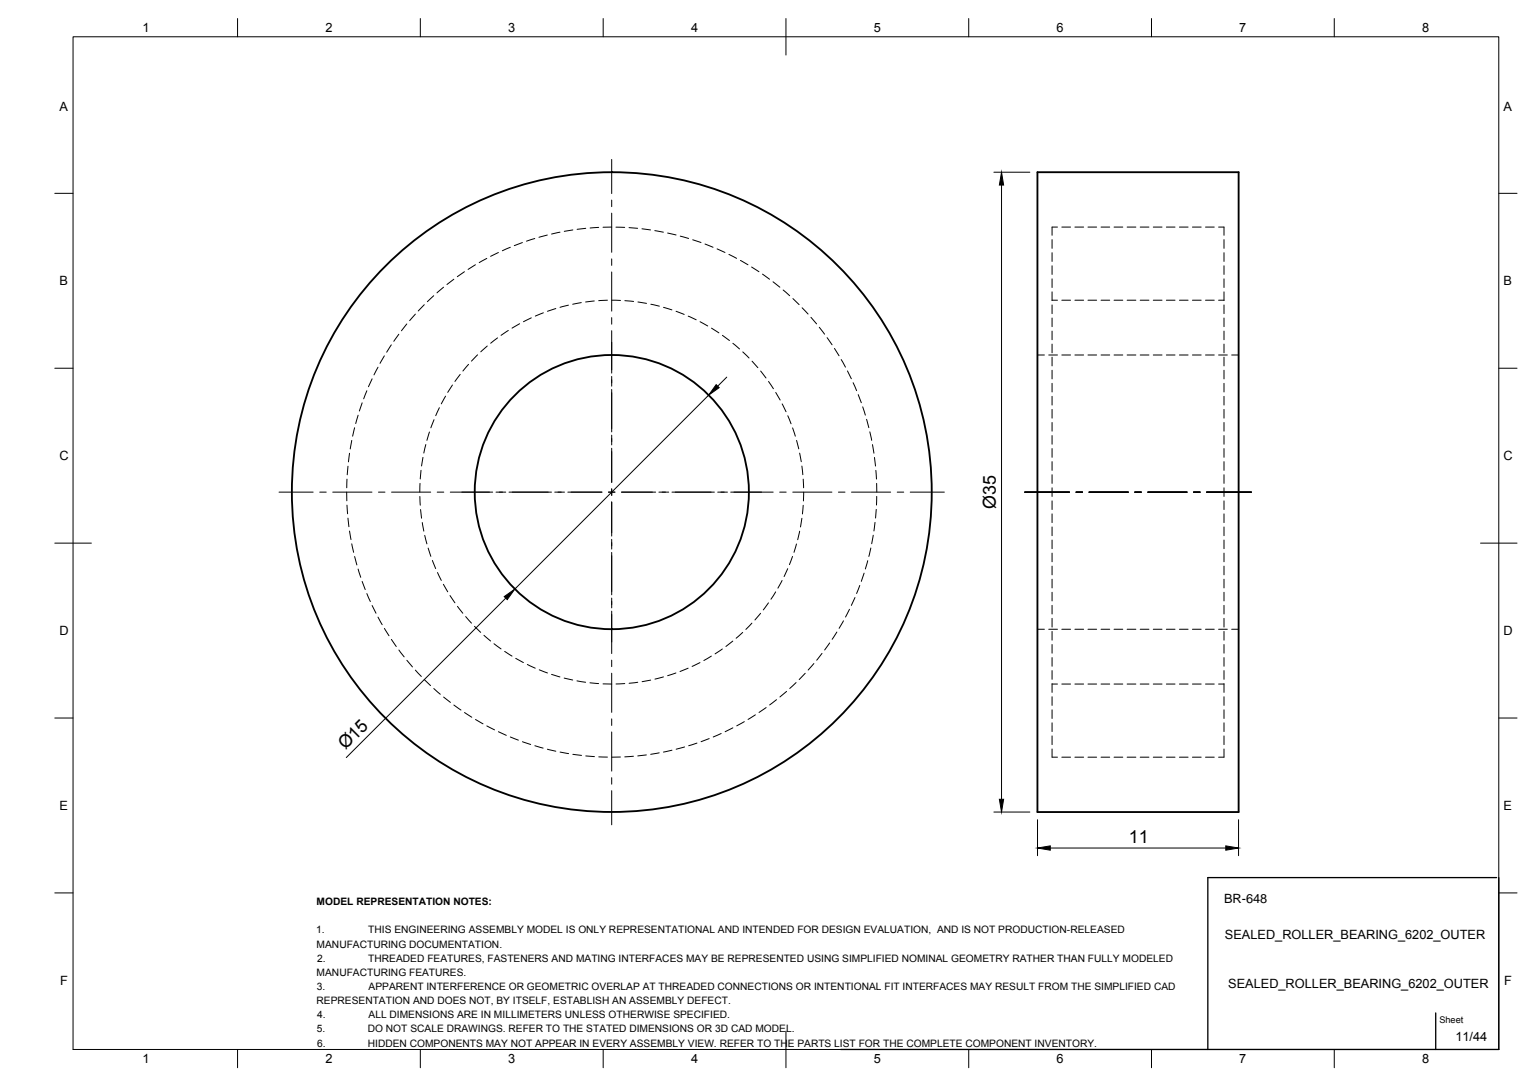
ISO-10303-21;
HEADER;
FILE_DESCRIPTION((''),'2;1');
FILE_NAME('SEALED_ROLLER_BEARING_6202_OUTER.step','2026-10-01T22:05:39-07:00',(''),(''),'','','');
FILE_SCHEMA (('AUTOMOTIVE_DESIGN { 1 0 10303 214 3 1 1 }'));
ENDSEC;
DATA;
#10=MECHANICAL_DESIGN_GEOMETRIC_PRESENTATION_REPRESENTATION('',(#611),#24628);
#485=ORIENTED_CLOSED_SHELL('',*,#13120,.F.) ;
#518=BREP_WITH_VOIDS('SEALED_ROLLER_BEARING_6202_OUTER',#13121,(#485)) ;
#527=SHAPE_REPRESENTATION_RELATIONSHIP('SRR','None',#24799,#569) ;
#569=ADVANCED_BREP_SHAPE_REPRESENTATION('',(#518),#24589) ;
#611=STYLED_ITEM('',(#25034),#518) ;
#839=FACE_BOUND('',#4045,.T.) ;
#840=FACE_BOUND('',#4047,.T.) ;
#841=FACE_BOUND('',#4051,.T.) ;
#842=FACE_BOUND('',#4054,.T.) ;
#1142=LINE('',#20621,#1978) ;
#1143=LINE('',#20623,#1979) ;
#1144=LINE('',#20632,#1980) ;
#1145=LINE('',#20637,#1981) ;
#1978=VECTOR('',#16365,1.05) ;
#1979=VECTOR('',#16368,1.45) ;
#1980=VECTOR('',#16379,1.75) ;
#1981=VECTOR('',#16386,0.75) ;
#2778=CYLINDRICAL_SURFACE('',#14068,1.05) ;
#2779=CYLINDRICAL_SURFACE('',#14069,1.45) ;
#2780=CYLINDRICAL_SURFACE('',#14073,1.75) ;
#2781=CYLINDRICAL_SURFACE('',#14077,0.75) ;
#3124=FACE_OUTER_BOUND('',#4044,.T.) ;
#3125=FACE_OUTER_BOUND('',#4046,.T.) ;
#3126=FACE_OUTER_BOUND('',#4048,.T.) ;
#3127=FACE_OUTER_BOUND('',#4049,.T.) ;
#3128=FACE_OUTER_BOUND('',#4050,.T.) ;
#3129=FACE_OUTER_BOUND('',#4052,.T.) ;
#3130=FACE_OUTER_BOUND('',#4053,.T.) ;
#3131=FACE_OUTER_BOUND('',#4055,.T.) ;
#4044=EDGE_LOOP('',(#9237)) ;
#4045=EDGE_LOOP('',(#9238)) ;
#4046=EDGE_LOOP('',(#9239)) ;
#4047=EDGE_LOOP('',(#9240)) ;
#4048=EDGE_LOOP('',(#9241,#9242,#9243,#9244)) ;
#4049=EDGE_LOOP('',(#9245,#9246,#9247,#9248)) ;
#4050=EDGE_LOOP('',(#9249)) ;
#4051=EDGE_LOOP('',(#9250)) ;
#4052=EDGE_LOOP('',(#9251,#9252,#9253,#9254)) ;
#4053=EDGE_LOOP('',(#9255)) ;
#4054=EDGE_LOOP('',(#9256)) ;
#4055=EDGE_LOOP('',(#9257,#9258,#9259,#9260)) ;
#4980=CIRCLE('',#14063,1.45) ;
#4981=CIRCLE('',#14064,1.05) ;
#4982=CIRCLE('',#14066,1.45) ;
#4983=CIRCLE('',#14067,1.05) ;
#4984=CIRCLE('',#14071,1.75) ;
#4985=CIRCLE('',#14072,0.75) ;
#4986=CIRCLE('',#14074,1.75) ;
#4987=CIRCLE('',#14076,0.75) ;
#5787=VERTEX_POINT('',#20611) ;
#5788=VERTEX_POINT('',#20613) ;
#5789=VERTEX_POINT('',#20616) ;
#5790=VERTEX_POINT('',#20618) ;
#5791=VERTEX_POINT('',#20625) ;
#5792=VERTEX_POINT('',#20627) ;
#5793=VERTEX_POINT('',#20630) ;
#5794=VERTEX_POINT('',#20634) ;
#7108=EDGE_CURVE('',#5787,#5787,#4980,.T.) ;
#7109=EDGE_CURVE('',#5788,#5788,#4981,.T.) ;
#7110=EDGE_CURVE('',#5789,#5789,#4982,.T.) ;
#7111=EDGE_CURVE('',#5790,#5790,#4983,.T.) ;
#7112=EDGE_CURVE('',#5788,#5790,#1142,.T.) ;
#7113=EDGE_CURVE('',#5789,#5787,#1143,.T.) ;
#7114=EDGE_CURVE('',#5791,#5791,#4984,.T.) ;
#7115=EDGE_CURVE('',#5792,#5792,#4985,.T.) ;
#7116=EDGE_CURVE('',#5793,#5793,#4986,.T.) ;
#7117=EDGE_CURVE('',#5793,#5791,#1144,.T.) ;
#7118=EDGE_CURVE('',#5794,#5794,#4987,.T.) ;
#7119=EDGE_CURVE('',#5792,#5794,#1145,.T.) ;
#9237=ORIENTED_EDGE('',*,*,#7108,.F.) ;
#9238=ORIENTED_EDGE('',*,*,#7109,.F.) ;
#9239=ORIENTED_EDGE('',*,*,#7110,.F.) ;
#9240=ORIENTED_EDGE('',*,*,#7111,.F.) ;
#9241=ORIENTED_EDGE('',*,*,#7109,.T.) ;
#9242=ORIENTED_EDGE('',*,*,#7112,.T.) ;
#9243=ORIENTED_EDGE('',*,*,#7111,.T.) ;
#9244=ORIENTED_EDGE('',*,*,#7112,.F.) ;
#9245=ORIENTED_EDGE('',*,*,#7110,.T.) ;
#9246=ORIENTED_EDGE('',*,*,#7113,.T.) ;
#9247=ORIENTED_EDGE('',*,*,#7108,.T.) ;
#9248=ORIENTED_EDGE('',*,*,#7113,.F.) ;
#9249=ORIENTED_EDGE('',*,*,#7114,.T.) ;
#9250=ORIENTED_EDGE('',*,*,#7115,.T.) ;
#9251=ORIENTED_EDGE('',*,*,#7116,.F.) ;
#9252=ORIENTED_EDGE('',*,*,#7117,.T.) ;
#9253=ORIENTED_EDGE('',*,*,#7114,.F.) ;
#9254=ORIENTED_EDGE('',*,*,#7117,.F.) ;
#9255=ORIENTED_EDGE('',*,*,#7116,.T.) ;
#9256=ORIENTED_EDGE('',*,*,#7118,.T.) ;
#9257=ORIENTED_EDGE('',*,*,#7115,.F.) ;
#9258=ORIENTED_EDGE('',*,*,#7119,.T.) ;
#9259=ORIENTED_EDGE('',*,*,#7118,.F.) ;
#9260=ORIENTED_EDGE('',*,*,#7119,.F.) ;
#12062=PLANE('',#14062) ;
#12063=PLANE('',#14065) ;
#12064=PLANE('',#14070) ;
#12065=PLANE('',#14075) ;
#12519=ADVANCED_FACE('',(#3124,#839),#12062,.T.) ;
#12520=ADVANCED_FACE('',(#3125,#840),#12063,.T.) ;
#12521=ADVANCED_FACE('',(#3126),#2778,.T.) ;
#12522=ADVANCED_FACE('',(#3127),#2779,.F.) ;
#12523=ADVANCED_FACE('',(#3128,#841),#12064,.T.) ;
#12524=ADVANCED_FACE('',(#3129),#2780,.T.) ;
#12525=ADVANCED_FACE('',(#3130,#842),#12065,.T.) ;
#12526=ADVANCED_FACE('',(#3131),#2781,.F.) ;
#13120=CLOSED_SHELL('',(#12519,#12520,#12521,#12522)) ;
#13121=CLOSED_SHELL('',(#12523,#12524,#12525,#12526)) ;
#14061=AXIS2_PLACEMENT_3D('',#20609,#16349,#16350) ;
#14062=AXIS2_PLACEMENT_3D('',#20610,#16351,#16352) ;
#14063=AXIS2_PLACEMENT_3D('',#20612,#16353,#16354) ;
#14064=AXIS2_PLACEMENT_3D('',#20614,#16355,#16356) ;
#14065=AXIS2_PLACEMENT_3D('',#20615,#16357,#16358) ;
#14066=AXIS2_PLACEMENT_3D('',#20617,#16359,#16360) ;
#14067=AXIS2_PLACEMENT_3D('',#20619,#16361,#16362) ;
#14068=AXIS2_PLACEMENT_3D('',#20620,#16363,#16364) ;
#14069=AXIS2_PLACEMENT_3D('',#20622,#16366,#16367) ;
#14070=AXIS2_PLACEMENT_3D('',#20624,#16369,#16370) ;
#14071=AXIS2_PLACEMENT_3D('',#20626,#16371,#16372) ;
#14072=AXIS2_PLACEMENT_3D('',#20628,#16373,#16374) ;
#14073=AXIS2_PLACEMENT_3D('',#20629,#16375,#16376) ;
#14074=AXIS2_PLACEMENT_3D('',#20631,#16377,#16378) ;
#14075=AXIS2_PLACEMENT_3D('',#20633,#16380,#16381) ;
#14076=AXIS2_PLACEMENT_3D('',#20635,#16382,#16383) ;
#14077=AXIS2_PLACEMENT_3D('',#20636,#16384,#16385) ;
#16349=DIRECTION('axis',(0.,0.,1.)) ;
#16350=DIRECTION('refdir',(1.,0.,0.)) ;
#16351=DIRECTION('center_axis',(0.,-1.,0.)) ;
#16352=DIRECTION('ref_axis',(-1.,0.,0.)) ;
#16353=DIRECTION('center_axis',(0.,1.,0.)) ;
#16354=DIRECTION('ref_axis',(1.,0.,0.)) ;
#16355=DIRECTION('center_axis',(0.,-1.,0.)) ;
#16356=DIRECTION('ref_axis',(1.,0.,0.)) ;
#16357=DIRECTION('center_axis',(0.,1.,0.)) ;
#16358=DIRECTION('ref_axis',(1.,0.,0.)) ;
#16359=DIRECTION('center_axis',(0.,-1.,0.)) ;
#16360=DIRECTION('ref_axis',(1.,0.,0.)) ;
#16361=DIRECTION('center_axis',(0.,1.,0.)) ;
#16362=DIRECTION('ref_axis',(1.,0.,0.)) ;
#16363=DIRECTION('center_axis',(0.,1.,0.)) ;
#16364=DIRECTION('ref_axis',(1.,0.,0.)) ;
#16365=DIRECTION('',(0.,-1.,0.)) ;
#16366=DIRECTION('center_axis',(0.,1.,0.)) ;
#16367=DIRECTION('ref_axis',(1.,0.,0.)) ;
#16368=DIRECTION('',(0.,1.,0.)) ;
#16369=DIRECTION('center_axis',(0.,-1.,0.)) ;
#16370=DIRECTION('ref_axis',(-1.,0.,0.)) ;
#16371=DIRECTION('center_axis',(0.,-1.,0.)) ;
#16372=DIRECTION('ref_axis',(1.,0.,0.)) ;
#16373=DIRECTION('center_axis',(0.,1.,0.)) ;
#16374=DIRECTION('ref_axis',(1.,0.,0.)) ;
#16375=DIRECTION('center_axis',(0.,1.,0.)) ;
#16376=DIRECTION('ref_axis',(1.,0.,0.)) ;
#16377=DIRECTION('center_axis',(0.,1.,0.)) ;
#16378=DIRECTION('ref_axis',(1.,0.,0.)) ;
#16379=DIRECTION('',(0.,-1.,0.)) ;
#16380=DIRECTION('center_axis',(0.,1.,0.)) ;
#16381=DIRECTION('ref_axis',(1.,0.,0.)) ;
#16382=DIRECTION('center_axis',(0.,-1.,0.)) ;
#16383=DIRECTION('ref_axis',(1.,0.,0.)) ;
#16384=DIRECTION('center_axis',(0.,1.,0.)) ;
#16385=DIRECTION('ref_axis',(1.,0.,0.)) ;
#16386=DIRECTION('',(0.,1.,0.)) ;
#20609=CARTESIAN_POINT('',(0.,0.,0.)) ;
#20610=CARTESIAN_POINT('Origin',(0.,-4.08,0.)) ;
#20611=CARTESIAN_POINT('',(-1.45,-4.08,1.77573785876366E-16)) ;
#20612=CARTESIAN_POINT('Origin',(0.,-4.08,0.)) ;
#20613=CARTESIAN_POINT('',(-1.05,-4.08,-1.28587913910472E-16)) ;
#20614=CARTESIAN_POINT('Origin',(0.,-4.08,0.)) ;
#20615=CARTESIAN_POINT('Origin',(0.,-5.02,0.)) ;
#20616=CARTESIAN_POINT('',(-1.45,-5.02,-1.77573785876366E-16)) ;
#20617=CARTESIAN_POINT('Origin',(0.,-5.02,0.)) ;
#20618=CARTESIAN_POINT('',(-1.05,-5.02,1.28587913910472E-16)) ;
#20619=CARTESIAN_POINT('Origin',(0.,-5.02,0.)) ;
#20620=CARTESIAN_POINT('Origin',(0.,-4.55,0.)) ;
#20621=CARTESIAN_POINT('',(-1.05,-4.55,1.28587913910472E-16)) ;
#20622=CARTESIAN_POINT('Origin',(0.,-4.55,0.)) ;
#20623=CARTESIAN_POINT('',(-1.45,-4.55,1.77573785876366E-16)) ;
#20624=CARTESIAN_POINT('Origin',(0.,-5.1,0.)) ;
#20625=CARTESIAN_POINT('',(-1.75,-5.1,2.14313189850787E-16)) ;
#20626=CARTESIAN_POINT('Origin',(0.,-5.1,0.)) ;
#20627=CARTESIAN_POINT('',(-0.75,-5.1,9.18485099360515E-17)) ;
#20628=CARTESIAN_POINT('Origin',(0.,-5.1,0.)) ;
#20629=CARTESIAN_POINT('Origin',(0.,-4.55,0.)) ;
#20630=CARTESIAN_POINT('',(-1.75,-4.,2.14313189850787E-16)) ;
#20631=CARTESIAN_POINT('Origin',(0.,-4.,0.)) ;
#20632=CARTESIAN_POINT('',(-1.75,-4.55,2.14313189850787E-16)) ;
#20633=CARTESIAN_POINT('Origin',(0.,-4.,0.)) ;
#20634=CARTESIAN_POINT('',(-0.75,-4.,-9.18485099360515E-17)) ;
#20635=CARTESIAN_POINT('Origin',(0.,-4.,0.)) ;
#20636=CARTESIAN_POINT('Origin',(0.,-4.55,0.)) ;
#20637=CARTESIAN_POINT('',(-0.75,-4.55,9.18485099360515E-17)) ;
#24541=UNCERTAINTY_MEASURE_WITH_UNIT(LENGTH_MEASURE(0.001),#24629,
'DISTANCE_ACCURACY_VALUE',
'Maximum model space distance between geometric entities at asserted c
onnectivities') ;
#24580=UNCERTAINTY_MEASURE_WITH_UNIT(LENGTH_MEASURE(0.001),#24629,
'DISTANCE_ACCURACY_VALUE',
'Maximum model space distance between geometric entities at asserted c
onnectivities') ;
#24589=(
GEOMETRIC_REPRESENTATION_CONTEXT(3)
GLOBAL_UNCERTAINTY_ASSIGNED_CONTEXT((#24541))
GLOBAL_UNIT_ASSIGNED_CONTEXT((#24629,#24631,#24632))
REPRESENTATION_CONTEXT('','3D')
) ;
#24628=(
GEOMETRIC_REPRESENTATION_CONTEXT(3)
GLOBAL_UNCERTAINTY_ASSIGNED_CONTEXT((#24580))
GLOBAL_UNIT_ASSIGNED_CONTEXT((#24629,#24631,#24632))
REPRESENTATION_CONTEXT('','3D')
) ;
#24629=(
LENGTH_UNIT()
NAMED_UNIT(*)
SI_UNIT(.CENTI.,.METRE.)
) ;
#24631=(
NAMED_UNIT(*)
PLANE_ANGLE_UNIT()
SI_UNIT($,.RADIAN.)
) ;
#24632=(
NAMED_UNIT(*)
SI_UNIT($,.STERADIAN.)
SOLID_ANGLE_UNIT()
) ;
#24641=SHAPE_DEFINITION_REPRESENTATION(#24688,#24799) ;
#24688=PRODUCT_DEFINITION_SHAPE('',$,#24847) ;
#24799=SHAPE_REPRESENTATION('',(#14061),#24589) ;
#24838=PRODUCT_DEFINITION_CONTEXT('part definition',#24981,'design') ;
#24847=PRODUCT_DEFINITION('SEALED_ROLLER_BEARING_6202_OUTER',
'SEALED_ROLLER_BEARING_6202_OUTER',#24894,#24838) ;
#24894=PRODUCT_DEFINITION_FORMATION('',$,#24991) ;
#24981=APPLICATION_CONTEXT(
'Core Data for Automotive Mechanical Design Process') ;
#24982=PRODUCT_CONTEXT('part definition',#24981,'mechanical') ;
#24991=PRODUCT('SEALED_ROLLER_BEARING_6202_OUTER',
'SEALED_ROLLER_BEARING_6202_OUTER',$,(#24982)) ;
#25034=PRESENTATION_STYLE_ASSIGNMENT((#25044)) ;
#25044=SURFACE_STYLE_USAGE(.BOTH.,#25054) ;
#25054=SURFACE_SIDE_STYLE('',(#25064)) ;
#25064=SURFACE_STYLE_FILL_AREA(#25074) ;
#25074=FILL_AREA_STYLE('Stainless Steel - Satin',(#25084)) ;
#25084=FILL_AREA_STYLE_COLOUR('Stainless Steel - Satin',#25094) ;
#25094=COLOUR_RGB('Stainless Steel - Satin', 0.31764706, 0.68627451, 0.89019608) ;
ENDSEC;
END-ISO-10303-21;
